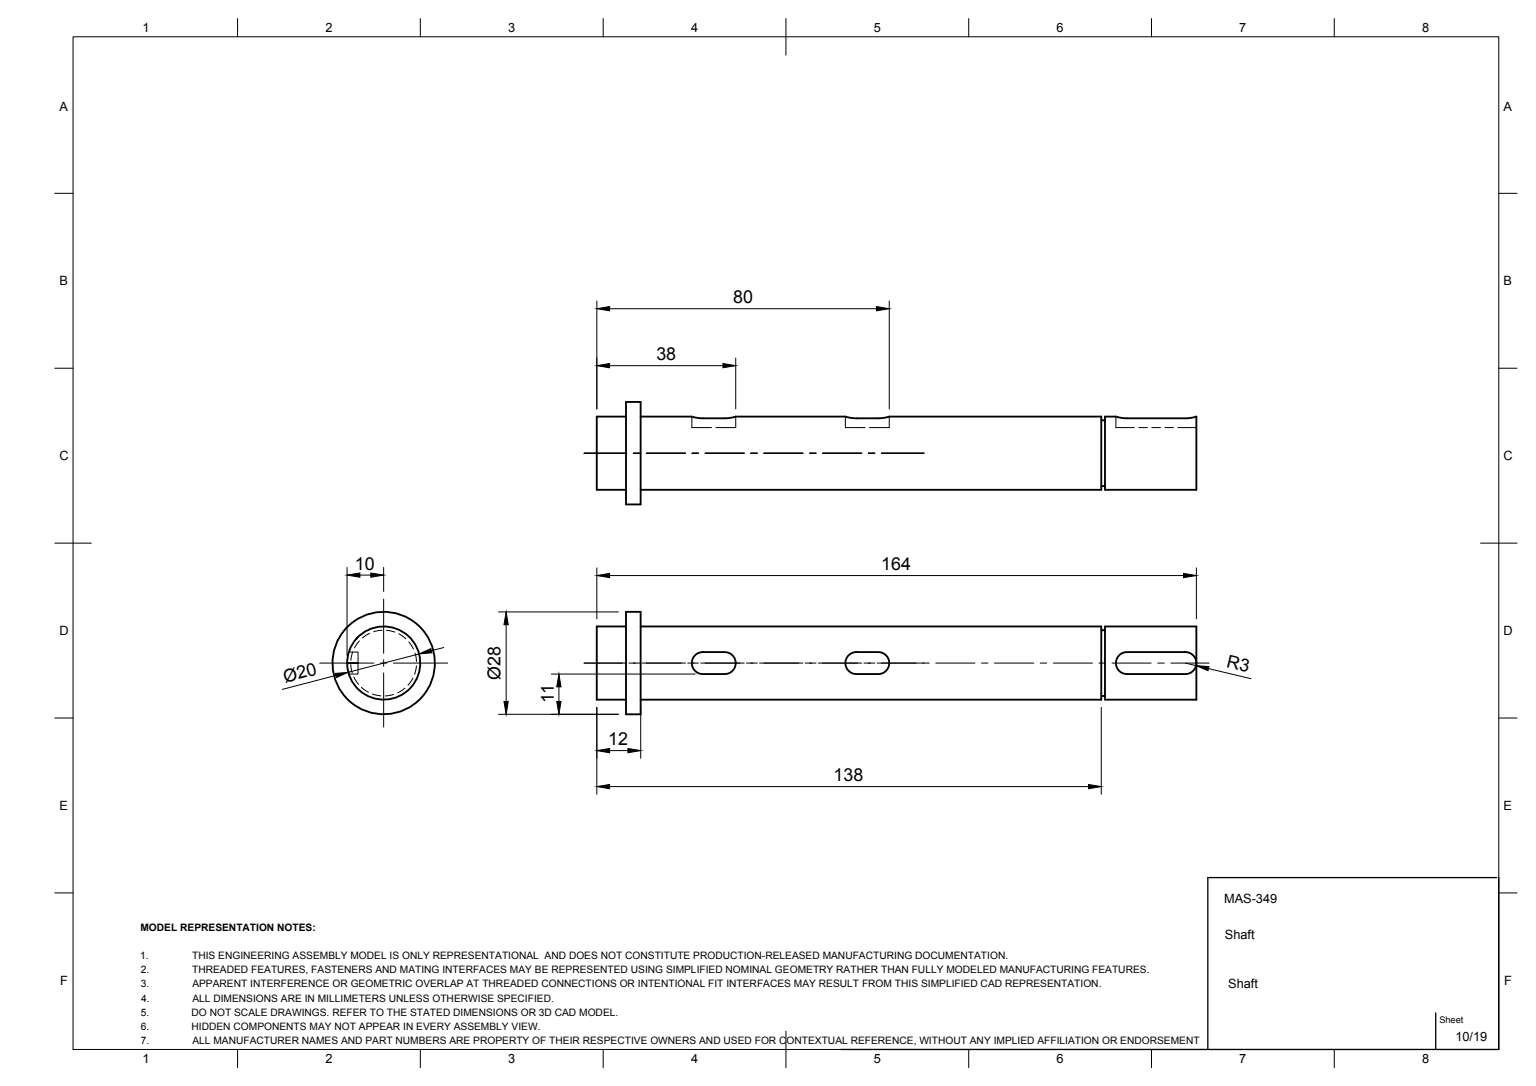
ISO-10303-21;
HEADER;
/* Generated by software containing ST-Developer
 * from STEP Tools, Inc. (www.steptools.com) 
 */

FILE_DESCRIPTION(
/* description */ ('Independent two-stage semi-open centrifugal-pump CAD. Shared impeller
s, open-machinable return casings, removable diaphragms, bronze wear/j
ournal rings, volume-preserving seal instances, retained keyed shaft, 
opposed mechanical face rings and partly threaded tie hardware. Native
 shaft rotation. Geometric topology/clearance only; flow/head/efficien
cy, pressure, cavitation, balance, preload, face loading and secondary
 seal fits/bonds, material/thermal/tolerance selection and life unassi
gned. External drive, coupling, anchors and piping bolts omitted.'),
/* implementation_level */ '2;1');

FILE_NAME(
/* name */ 'Shaft.step',
/* time_stamp */ '2026-11-08T18:06:32-08:00',
/* author */ (''),
/* organization */ (''),
/* preprocessor_version */ 'ST-DEVELOPER v20.2',
/* originating_system */ 'Autodesk Translation Framework v15.17.0.0',
/* authorisation */ '');

FILE_SCHEMA (('AUTOMOTIVE_DESIGN { 1 0 10303 214 3 1 1 }'));
ENDSEC;

DATA;
#10=MECHANICAL_DESIGN_GEOMETRIC_PRESENTATION_REPRESENTATION('',(#400),#16687);
#311=B_SPLINE_CURVE_WITH_KNOTS('',3,(#14886,#14887,#14888,#14889,#14890,
#14891,#14892,#14893,#14894,#14895),.UNSPECIFIED.,.F.,.F.,(4,2,2,2,4),(-0.455064911568752,
-0.341315631981151,-0.227566352393549,-0.113783176196775,0.),
 .UNSPECIFIED.);
#312=B_SPLINE_CURVE_WITH_KNOTS('',3,(#14898,#14899,#14900,#14901,#14902,
#14903,#14904,#14905,#14906,#14907),.UNSPECIFIED.,.F.,.F.,(4,2,2,2,4),(-0.910129823137504,
-0.796346646940729,-0.682563470743954,-0.568814191156353,-0.455064911568752),
 .UNSPECIFIED.);
#313=B_SPLINE_CURVE_WITH_KNOTS('',3,(#14920,#14921,#14922,#14923,#14924,
#14925,#14926,#14927,#14928,#14929,#14930,#14931,#14932,#14933,#14934,#14935,
#14936,#14937),.UNSPECIFIED.,.F.,.F.,(4,2,2,2,2,2,2,2,4),(0.,0.113783176196775,
0.227566352393549,0.34131563198115,0.455064911568751,0.568814191156352,
0.682563470743952,0.796346646940728,0.910129823137503),.UNSPECIFIED.);
#314=B_SPLINE_CURVE_WITH_KNOTS('',3,(#14963,#14964,#14965,#14966,#14967,
#14968,#14969,#14970,#14971,#14972,#14973,#14974,#14975,#14976,#14977,#14978,
#14979,#14980),.UNSPECIFIED.,.F.,.F.,(4,2,2,2,2,2,2,2,4),(-0.910129823137502,
-0.796346646940727,-0.682563470743952,-0.568814191156352,-0.455064911568751,
-0.34131563198115,-0.227566352393549,-0.113783176196775,0.),
 .UNSPECIFIED.);
#315=B_SPLINE_CURVE_WITH_KNOTS('',3,(#14991,#14992,#14993,#14994,#14995,
#14996,#14997,#14998,#14999,#15000,#15001,#15002,#15003,#15004,#15005,#15006,
#15007,#15008),.UNSPECIFIED.,.F.,.F.,(4,2,2,2,2,2,2,2,4),(0.,0.113783176196775,
0.227566352393549,0.34131563198115,0.455064911568751,0.568814191156351,
0.682563470743952,0.796346646940727,0.910129823137502),.UNSPECIFIED.);
#316=B_SPLINE_CURVE_WITH_KNOTS('',3,(#15022,#15023,#15024,#15025,#15026,
#15027,#15028,#15029,#15030,#15031,#15032,#15033,#15034,#15035,#15036,#15037,
#15038,#15039),.UNSPECIFIED.,.F.,.F.,(4,2,2,2,2,2,2,2,4),(-0.910129823137502,
-0.796346646940727,-0.682563470743952,-0.568814191156352,-0.455064911568751,
-0.34131563198115,-0.22756635239355,-0.113783176196775,0.),
 .UNSPECIFIED.);
#317=B_SPLINE_CURVE_WITH_KNOTS('',3,(#15050,#15051,#15052,#15053,#15054,
#15055,#15056,#15057,#15058,#15059,#15060,#15061,#15062,#15063,#15064,#15065,
#15066,#15067),.UNSPECIFIED.,.F.,.F.,(4,2,2,2,2,2,2,2,4),(0.,0.113783176196775,
0.22756635239355,0.341315631981151,0.455064911568751,0.568814191156352,
0.682563470743953,0.796346646940727,0.910129823137502),.UNSPECIFIED.);
#362=SHAPE_REPRESENTATION_RELATIONSHIP('SRR','None',#16771,#381);
#381=ADVANCED_BREP_SHAPE_REPRESENTATION('',(#419),#16675);
#400=STYLED_ITEM('',(#16873),#419);
#419=MANIFOLD_SOLID_BREP('Body1',#6119);
#529=FACE_BOUND('',#1395,.T.);
#530=FACE_BOUND('',#1397,.T.);
#531=FACE_BOUND('',#1399,.T.);
#532=FACE_BOUND('',#1401,.T.);
#533=FACE_BOUND('',#1405,.T.);
#534=FACE_BOUND('',#1406,.T.);
#636=PLANE('',#6783);
#637=PLANE('',#6786);
#638=PLANE('',#6787);
#639=PLANE('',#6792);
#640=PLANE('',#6795);
#641=PLANE('',#6798);
#642=PLANE('',#6799);
#643=PLANE('',#6802);
#644=PLANE('',#6805);
#645=PLANE('',#6809);
#646=PLANE('',#6811);
#647=PLANE('',#6812);
#648=PLANE('',#6815);
#649=PLANE('',#6822);
#650=PLANE('',#6823);
#931=FACE_OUTER_BOUND('',#1376,.T.);
#932=FACE_OUTER_BOUND('',#1377,.T.);
#933=FACE_OUTER_BOUND('',#1378,.T.);
#934=FACE_OUTER_BOUND('',#1379,.T.);
#935=FACE_OUTER_BOUND('',#1380,.T.);
#936=FACE_OUTER_BOUND('',#1381,.T.);
#937=FACE_OUTER_BOUND('',#1382,.T.);
#938=FACE_OUTER_BOUND('',#1383,.T.);
#939=FACE_OUTER_BOUND('',#1384,.T.);
#940=FACE_OUTER_BOUND('',#1385,.T.);
#941=FACE_OUTER_BOUND('',#1386,.T.);
#942=FACE_OUTER_BOUND('',#1387,.T.);
#943=FACE_OUTER_BOUND('',#1388,.T.);
#944=FACE_OUTER_BOUND('',#1389,.T.);
#945=FACE_OUTER_BOUND('',#1390,.T.);
#946=FACE_OUTER_BOUND('',#1391,.T.);
#947=FACE_OUTER_BOUND('',#1392,.T.);
#948=FACE_OUTER_BOUND('',#1393,.T.);
#949=FACE_OUTER_BOUND('',#1394,.T.);
#950=FACE_OUTER_BOUND('',#1396,.T.);
#951=FACE_OUTER_BOUND('',#1398,.T.);
#952=FACE_OUTER_BOUND('',#1400,.T.);
#953=FACE_OUTER_BOUND('',#1402,.T.);
#954=FACE_OUTER_BOUND('',#1403,.T.);
#955=FACE_OUTER_BOUND('',#1404,.T.);
#956=FACE_OUTER_BOUND('',#1407,.T.);
#957=FACE_OUTER_BOUND('',#1408,.T.);
#1376=EDGE_LOOP('',(#5145,#5146,#5147,#5148));
#1377=EDGE_LOOP('',(#5149,#5150,#5151,#5152));
#1378=EDGE_LOOP('',(#5153,#5154,#5155,#5156));
#1379=EDGE_LOOP('',(#5157,#5158,#5159,#5160));
#1380=EDGE_LOOP('',(#5161,#5162,#5163,#5164));
#1381=EDGE_LOOP('',(#5165,#5166,#5167,#5168,#5169));
#1382=EDGE_LOOP('',(#5170,#5171,#5172,#5173,#5174,#5175,#5176,#5177,#5178,
#5179));
#1383=EDGE_LOOP('',(#5180,#5181,#5182,#5183));
#1384=EDGE_LOOP('',(#5184,#5185,#5186,#5187));
#1385=EDGE_LOOP('',(#5188,#5189,#5190,#5191));
#1386=EDGE_LOOP('',(#5192,#5193,#5194,#5195));
#1387=EDGE_LOOP('',(#5196,#5197,#5198,#5199));
#1388=EDGE_LOOP('',(#5200,#5201,#5202,#5203));
#1389=EDGE_LOOP('',(#5204,#5205,#5206,#5207));
#1390=EDGE_LOOP('',(#5208,#5209,#5210,#5211));
#1391=EDGE_LOOP('',(#5212,#5213,#5214,#5215));
#1392=EDGE_LOOP('',(#5216,#5217,#5218,#5219));
#1393=EDGE_LOOP('',(#5220,#5221,#5222,#5223));
#1394=EDGE_LOOP('',(#5224));
#1395=EDGE_LOOP('',(#5225));
#1396=EDGE_LOOP('',(#5226));
#1397=EDGE_LOOP('',(#5227));
#1398=EDGE_LOOP('',(#5228));
#1399=EDGE_LOOP('',(#5229));
#1400=EDGE_LOOP('',(#5230));
#1401=EDGE_LOOP('',(#5231));
#1402=EDGE_LOOP('',(#5232,#5233,#5234,#5235));
#1403=EDGE_LOOP('',(#5236,#5237,#5238,#5239));
#1404=EDGE_LOOP('',(#5240,#5241,#5242,#5243));
#1405=EDGE_LOOP('',(#5244,#5245,#5246,#5247));
#1406=EDGE_LOOP('',(#5248,#5249,#5250,#5251));
#1407=EDGE_LOOP('',(#5252,#5253,#5254,#5255));
#1408=EDGE_LOOP('',(#5256));
#1773=LINE('',#14881,#2142);
#1774=LINE('',#14885,#2143);
#1775=LINE('',#14909,#2144);
#1776=LINE('',#14911,#2145);
#1777=LINE('',#14914,#2146);
#1778=LINE('',#14916,#2147);
#1779=LINE('',#14917,#2148);
#1780=LINE('',#14940,#2149);
#1781=LINE('',#14942,#2150);
#1782=LINE('',#14943,#2151);
#1783=LINE('',#14950,#2152);
#1784=LINE('',#14955,#2153);
#1785=LINE('',#14957,#2154);
#1786=LINE('',#14959,#2155);
#1787=LINE('',#14960,#2156);
#1788=LINE('',#14983,#2157);
#1789=LINE('',#14986,#2158);
#1790=LINE('',#14988,#2159);
#1791=LINE('',#14989,#2160);
#1792=LINE('',#15014,#2161);
#1793=LINE('',#15016,#2162);
#1794=LINE('',#15018,#2163);
#1795=LINE('',#15019,#2164);
#1796=LINE('',#15042,#2165);
#1797=LINE('',#15045,#2166);
#1798=LINE('',#15047,#2167);
#1799=LINE('',#15048,#2168);
#1800=LINE('',#15074,#2169);
#1801=LINE('',#15091,#2170);
#1802=LINE('',#15094,#2171);
#1803=LINE('',#15097,#2172);
#2142=VECTOR('',#8137,1.);
#2143=VECTOR('',#8140,1.);
#2144=VECTOR('',#8143,1.);
#2145=VECTOR('',#8146,1.);
#2146=VECTOR('',#8149,1.);
#2147=VECTOR('',#8150,1.);
#2148=VECTOR('',#8151,1.);
#2149=VECTOR('',#8156,1.);
#2150=VECTOR('',#8159,1.);
#2151=VECTOR('',#8160,1.);
#2152=VECTOR('',#8169,1.);
#2153=VECTOR('',#8174,1.);
#2154=VECTOR('',#8175,1.);
#2155=VECTOR('',#8176,1.);
#2156=VECTOR('',#8177,1.);
#2157=VECTOR('',#8182,1.);
#2158=VECTOR('',#8185,1.);
#2159=VECTOR('',#8186,1.);
#2160=VECTOR('',#8187,1.);
#2161=VECTOR('',#8196,1.);
#2162=VECTOR('',#8197,1.);
#2163=VECTOR('',#8198,1.);
#2164=VECTOR('',#8199,1.);
#2165=VECTOR('',#8204,1.);
#2166=VECTOR('',#8207,1.);
#2167=VECTOR('',#8208,1.);
#2168=VECTOR('',#8209,1.);
#2169=VECTOR('',#8220,0.9);
#2170=VECTOR('',#8243,1.4);
#2171=VECTOR('',#8246,1.);
#2172=VECTOR('',#8251,1.);
#2432=CIRCLE('',#6780,0.3);
#2433=CIRCLE('',#6782,0.3);
#2434=CIRCLE('',#6785,0.3);
#2435=CIRCLE('',#6789,1.);
#2436=CIRCLE('',#6790,1.);
#2437=CIRCLE('',#6791,1.);
#2438=CIRCLE('',#6794,0.3);
#2439=CIRCLE('',#6797,0.3);
#2440=CIRCLE('',#6801,0.3);
#2441=CIRCLE('',#6804,0.3);
#2442=CIRCLE('',#6807,0.9);
#2443=CIRCLE('',#6808,0.9);
#2444=CIRCLE('',#6810,1.);
#2445=CIRCLE('',#6813,1.4);
#2446=CIRCLE('',#6814,1.);
#2447=CIRCLE('',#6816,1.4);
#2448=CIRCLE('',#6817,1.);
#2449=CIRCLE('',#6820,1.);
#2917=VERTEX_POINT('',#14879);
#2918=VERTEX_POINT('',#14880);
#2919=VERTEX_POINT('',#14882);
#2920=VERTEX_POINT('',#14884);
#2921=VERTEX_POINT('',#14897);
#2922=VERTEX_POINT('',#14908);
#2923=VERTEX_POINT('',#14913);
#2924=VERTEX_POINT('',#14915);
#2925=VERTEX_POINT('',#14919);
#2926=VERTEX_POINT('',#14938);
#2927=VERTEX_POINT('',#14946);
#2928=VERTEX_POINT('',#14949);
#2929=VERTEX_POINT('',#14953);
#2930=VERTEX_POINT('',#14954);
#2931=VERTEX_POINT('',#14956);
#2932=VERTEX_POINT('',#14958);
#2933=VERTEX_POINT('',#14962);
#2934=VERTEX_POINT('',#14981);
#2935=VERTEX_POINT('',#14985);
#2936=VERTEX_POINT('',#14987);
#2937=VERTEX_POINT('',#15012);
#2938=VERTEX_POINT('',#15013);
#2939=VERTEX_POINT('',#15015);
#2940=VERTEX_POINT('',#15017);
#2941=VERTEX_POINT('',#15021);
#2942=VERTEX_POINT('',#15040);
#2943=VERTEX_POINT('',#15044);
#2944=VERTEX_POINT('',#15046);
#2945=VERTEX_POINT('',#15071);
#2946=VERTEX_POINT('',#15073);
#2947=VERTEX_POINT('',#15077);
#2948=VERTEX_POINT('',#15081);
#2949=VERTEX_POINT('',#15083);
#2950=VERTEX_POINT('',#15086);
#2951=VERTEX_POINT('',#15088);
#2952=VERTEX_POINT('',#15093);
#3682=EDGE_CURVE('',#2917,#2918,#1773,.T.);
#3683=EDGE_CURVE('',#2919,#2917,#2432,.T.);
#3684=EDGE_CURVE('',#2919,#2920,#1774,.T.);
#3685=EDGE_CURVE('',#2918,#2920,#311,.T.);
#3686=EDGE_CURVE('',#2921,#2918,#312,.T.);
#3687=EDGE_CURVE('',#2922,#2921,#1775,.T.);
#3688=EDGE_CURVE('',#2917,#2922,#2433,.T.);
#3689=EDGE_CURVE('',#2917,#2918,#1776,.T.);
#3690=EDGE_CURVE('',#2920,#2923,#1777,.T.);
#3691=EDGE_CURVE('',#2919,#2924,#1778,.T.);
#3692=EDGE_CURVE('',#2924,#2923,#1779,.T.);
#3693=EDGE_CURVE('',#2923,#2925,#313,.T.);
#3694=EDGE_CURVE('',#2926,#2924,#2434,.T.);
#3695=EDGE_CURVE('',#2926,#2925,#1780,.T.);
#3696=EDGE_CURVE('',#2925,#2921,#1781,.T.);
#3697=EDGE_CURVE('',#2926,#2922,#1782,.T.);
#3698=EDGE_CURVE('',#2918,#2927,#2435,.T.);
#3699=EDGE_CURVE('',#2927,#2918,#2436,.T.);
#3700=EDGE_CURVE('',#2927,#2928,#1783,.T.);
#3701=EDGE_CURVE('',#2928,#2928,#2437,.T.);
#3702=EDGE_CURVE('',#2929,#2930,#1784,.T.);
#3703=EDGE_CURVE('',#2931,#2929,#1785,.T.);
#3704=EDGE_CURVE('',#2931,#2932,#1786,.T.);
#3705=EDGE_CURVE('',#2932,#2930,#1787,.T.);
#3706=EDGE_CURVE('',#2930,#2933,#314,.T.);
#3707=EDGE_CURVE('',#2934,#2932,#2438,.T.);
#3708=EDGE_CURVE('',#2934,#2933,#1788,.T.);
#3709=EDGE_CURVE('',#2933,#2935,#1789,.T.);
#3710=EDGE_CURVE('',#2934,#2936,#1790,.T.);
#3711=EDGE_CURVE('',#2936,#2935,#1791,.T.);
#3712=EDGE_CURVE('',#2935,#2929,#315,.T.);
#3713=EDGE_CURVE('',#2931,#2936,#2439,.T.);
#3714=EDGE_CURVE('',#2937,#2938,#1792,.T.);
#3715=EDGE_CURVE('',#2939,#2937,#1793,.T.);
#3716=EDGE_CURVE('',#2939,#2940,#1794,.T.);
#3717=EDGE_CURVE('',#2940,#2938,#1795,.T.);
#3718=EDGE_CURVE('',#2938,#2941,#316,.T.);
#3719=EDGE_CURVE('',#2942,#2940,#2440,.T.);
#3720=EDGE_CURVE('',#2942,#2941,#1796,.T.);
#3721=EDGE_CURVE('',#2941,#2943,#1797,.T.);
#3722=EDGE_CURVE('',#2942,#2944,#1798,.T.);
#3723=EDGE_CURVE('',#2944,#2943,#1799,.T.);
#3724=EDGE_CURVE('',#2943,#2937,#317,.T.);
#3725=EDGE_CURVE('',#2939,#2944,#2441,.T.);
#3726=EDGE_CURVE('',#2945,#2945,#2442,.T.);
#3727=EDGE_CURVE('',#2945,#2946,#1800,.T.);
#3728=EDGE_CURVE('',#2946,#2946,#2443,.T.);
#3729=EDGE_CURVE('',#2947,#2947,#2444,.T.);
#3730=EDGE_CURVE('',#2948,#2948,#2445,.T.);
#3731=EDGE_CURVE('',#2949,#2949,#2446,.T.);
#3732=EDGE_CURVE('',#2950,#2950,#2447,.T.);
#3733=EDGE_CURVE('',#2951,#2951,#2448,.T.);
#3734=EDGE_CURVE('',#2948,#2950,#1801,.T.);
#3735=EDGE_CURVE('',#2951,#2952,#1802,.T.);
#3736=EDGE_CURVE('',#2952,#2952,#2449,.T.);
#3737=EDGE_CURVE('',#2947,#2949,#1803,.T.);
#5145=ORIENTED_EDGE('',*,*,#3682,.F.);
#5146=ORIENTED_EDGE('',*,*,#3683,.F.);
#5147=ORIENTED_EDGE('',*,*,#3684,.T.);
#5148=ORIENTED_EDGE('',*,*,#3685,.F.);
#5149=ORIENTED_EDGE('',*,*,#3686,.F.);
#5150=ORIENTED_EDGE('',*,*,#3687,.F.);
#5151=ORIENTED_EDGE('',*,*,#3688,.F.);
#5152=ORIENTED_EDGE('',*,*,#3689,.T.);
#5153=ORIENTED_EDGE('',*,*,#3690,.F.);
#5154=ORIENTED_EDGE('',*,*,#3684,.F.);
#5155=ORIENTED_EDGE('',*,*,#3691,.T.);
#5156=ORIENTED_EDGE('',*,*,#3692,.T.);
#5157=ORIENTED_EDGE('',*,*,#3693,.F.);
#5158=ORIENTED_EDGE('',*,*,#3692,.F.);
#5159=ORIENTED_EDGE('',*,*,#3694,.F.);
#5160=ORIENTED_EDGE('',*,*,#3695,.T.);
#5161=ORIENTED_EDGE('',*,*,#3696,.F.);
#5162=ORIENTED_EDGE('',*,*,#3695,.F.);
#5163=ORIENTED_EDGE('',*,*,#3697,.T.);
#5164=ORIENTED_EDGE('',*,*,#3687,.T.);
#5165=ORIENTED_EDGE('',*,*,#3683,.T.);
#5166=ORIENTED_EDGE('',*,*,#3688,.T.);
#5167=ORIENTED_EDGE('',*,*,#3697,.F.);
#5168=ORIENTED_EDGE('',*,*,#3694,.T.);
#5169=ORIENTED_EDGE('',*,*,#3691,.F.);
#5170=ORIENTED_EDGE('',*,*,#3698,.F.);
#5171=ORIENTED_EDGE('',*,*,#3685,.T.);
#5172=ORIENTED_EDGE('',*,*,#3690,.T.);
#5173=ORIENTED_EDGE('',*,*,#3693,.T.);
#5174=ORIENTED_EDGE('',*,*,#3696,.T.);
#5175=ORIENTED_EDGE('',*,*,#3686,.T.);
#5176=ORIENTED_EDGE('',*,*,#3699,.F.);
#5177=ORIENTED_EDGE('',*,*,#3700,.T.);
#5178=ORIENTED_EDGE('',*,*,#3701,.T.);
#5179=ORIENTED_EDGE('',*,*,#3700,.F.);
#5180=ORIENTED_EDGE('',*,*,#3702,.F.);
#5181=ORIENTED_EDGE('',*,*,#3703,.F.);
#5182=ORIENTED_EDGE('',*,*,#3704,.T.);
#5183=ORIENTED_EDGE('',*,*,#3705,.T.);
#5184=ORIENTED_EDGE('',*,*,#3706,.F.);
#5185=ORIENTED_EDGE('',*,*,#3705,.F.);
#5186=ORIENTED_EDGE('',*,*,#3707,.F.);
#5187=ORIENTED_EDGE('',*,*,#3708,.T.);
#5188=ORIENTED_EDGE('',*,*,#3709,.F.);
#5189=ORIENTED_EDGE('',*,*,#3708,.F.);
#5190=ORIENTED_EDGE('',*,*,#3710,.T.);
#5191=ORIENTED_EDGE('',*,*,#3711,.T.);
#5192=ORIENTED_EDGE('',*,*,#3712,.F.);
#5193=ORIENTED_EDGE('',*,*,#3711,.F.);
#5194=ORIENTED_EDGE('',*,*,#3713,.F.);
#5195=ORIENTED_EDGE('',*,*,#3703,.T.);
#5196=ORIENTED_EDGE('',*,*,#3707,.T.);
#5197=ORIENTED_EDGE('',*,*,#3704,.F.);
#5198=ORIENTED_EDGE('',*,*,#3713,.T.);
#5199=ORIENTED_EDGE('',*,*,#3710,.F.);
#5200=ORIENTED_EDGE('',*,*,#3714,.F.);
#5201=ORIENTED_EDGE('',*,*,#3715,.F.);
#5202=ORIENTED_EDGE('',*,*,#3716,.T.);
#5203=ORIENTED_EDGE('',*,*,#3717,.T.);
#5204=ORIENTED_EDGE('',*,*,#3718,.F.);
#5205=ORIENTED_EDGE('',*,*,#3717,.F.);
#5206=ORIENTED_EDGE('',*,*,#3719,.F.);
#5207=ORIENTED_EDGE('',*,*,#3720,.T.);
#5208=ORIENTED_EDGE('',*,*,#3721,.F.);
#5209=ORIENTED_EDGE('',*,*,#3720,.F.);
#5210=ORIENTED_EDGE('',*,*,#3722,.T.);
#5211=ORIENTED_EDGE('',*,*,#3723,.T.);
#5212=ORIENTED_EDGE('',*,*,#3724,.F.);
#5213=ORIENTED_EDGE('',*,*,#3723,.F.);
#5214=ORIENTED_EDGE('',*,*,#3725,.F.);
#5215=ORIENTED_EDGE('',*,*,#3715,.T.);
#5216=ORIENTED_EDGE('',*,*,#3719,.T.);
#5217=ORIENTED_EDGE('',*,*,#3716,.F.);
#5218=ORIENTED_EDGE('',*,*,#3725,.T.);
#5219=ORIENTED_EDGE('',*,*,#3722,.F.);
#5220=ORIENTED_EDGE('',*,*,#3726,.T.);
#5221=ORIENTED_EDGE('',*,*,#3727,.T.);
#5222=ORIENTED_EDGE('',*,*,#3728,.F.);
#5223=ORIENTED_EDGE('',*,*,#3727,.F.);
#5224=ORIENTED_EDGE('',*,*,#3729,.F.);
#5225=ORIENTED_EDGE('',*,*,#3726,.F.);
#5226=ORIENTED_EDGE('',*,*,#3701,.F.);
#5227=ORIENTED_EDGE('',*,*,#3728,.T.);
#5228=ORIENTED_EDGE('',*,*,#3730,.T.);
#5229=ORIENTED_EDGE('',*,*,#3731,.F.);
#5230=ORIENTED_EDGE('',*,*,#3732,.F.);
#5231=ORIENTED_EDGE('',*,*,#3733,.F.);
#5232=ORIENTED_EDGE('',*,*,#3730,.F.);
#5233=ORIENTED_EDGE('',*,*,#3734,.T.);
#5234=ORIENTED_EDGE('',*,*,#3732,.T.);
#5235=ORIENTED_EDGE('',*,*,#3734,.F.);
#5236=ORIENTED_EDGE('',*,*,#3733,.T.);
#5237=ORIENTED_EDGE('',*,*,#3735,.T.);
#5238=ORIENTED_EDGE('',*,*,#3736,.T.);
#5239=ORIENTED_EDGE('',*,*,#3735,.F.);
#5240=ORIENTED_EDGE('',*,*,#3729,.T.);
#5241=ORIENTED_EDGE('',*,*,#3737,.T.);
#5242=ORIENTED_EDGE('',*,*,#3731,.T.);
#5243=ORIENTED_EDGE('',*,*,#3737,.F.);
#5244=ORIENTED_EDGE('',*,*,#3709,.T.);
#5245=ORIENTED_EDGE('',*,*,#3712,.T.);
#5246=ORIENTED_EDGE('',*,*,#3702,.T.);
#5247=ORIENTED_EDGE('',*,*,#3706,.T.);
#5248=ORIENTED_EDGE('',*,*,#3721,.T.);
#5249=ORIENTED_EDGE('',*,*,#3724,.T.);
#5250=ORIENTED_EDGE('',*,*,#3714,.T.);
#5251=ORIENTED_EDGE('',*,*,#3718,.T.);
#5252=ORIENTED_EDGE('',*,*,#3698,.T.);
#5253=ORIENTED_EDGE('',*,*,#3699,.T.);
#5254=ORIENTED_EDGE('',*,*,#3689,.F.);
#5255=ORIENTED_EDGE('',*,*,#3682,.T.);
#5256=ORIENTED_EDGE('',*,*,#3736,.F.);
#5716=CYLINDRICAL_SURFACE('',#6779,0.3);
#5717=CYLINDRICAL_SURFACE('',#6781,0.3);
#5718=CYLINDRICAL_SURFACE('',#6784,0.3);
#5719=CYLINDRICAL_SURFACE('',#6788,1.);
#5720=CYLINDRICAL_SURFACE('',#6793,0.3);
#5721=CYLINDRICAL_SURFACE('',#6796,0.3);
#5722=CYLINDRICAL_SURFACE('',#6800,0.3);
#5723=CYLINDRICAL_SURFACE('',#6803,0.3);
#5724=CYLINDRICAL_SURFACE('',#6806,0.9);
#5725=CYLINDRICAL_SURFACE('',#6818,1.4);
#5726=CYLINDRICAL_SURFACE('',#6819,1.);
#5727=CYLINDRICAL_SURFACE('',#6821,1.);
#6010=ADVANCED_FACE('',(#931),#5716,.F.);
#6011=ADVANCED_FACE('',(#932),#5717,.F.);
#6012=ADVANCED_FACE('',(#933),#636,.F.);
#6013=ADVANCED_FACE('',(#934),#5718,.F.);
#6014=ADVANCED_FACE('',(#935),#637,.F.);
#6015=ADVANCED_FACE('',(#936),#638,.T.);
#6016=ADVANCED_FACE('',(#937),#5719,.T.);
#6017=ADVANCED_FACE('',(#938),#639,.F.);
#6018=ADVANCED_FACE('',(#939),#5720,.F.);
#6019=ADVANCED_FACE('',(#940),#640,.F.);
#6020=ADVANCED_FACE('',(#941),#5721,.F.);
#6021=ADVANCED_FACE('',(#942),#641,.T.);
#6022=ADVANCED_FACE('',(#943),#642,.F.);
#6023=ADVANCED_FACE('',(#944),#5722,.F.);
#6024=ADVANCED_FACE('',(#945),#643,.F.);
#6025=ADVANCED_FACE('',(#946),#5723,.F.);
#6026=ADVANCED_FACE('',(#947),#644,.T.);
#6027=ADVANCED_FACE('',(#948),#5724,.T.);
#6028=ADVANCED_FACE('',(#949,#529),#645,.F.);
#6029=ADVANCED_FACE('',(#950,#530),#646,.F.);
#6030=ADVANCED_FACE('',(#951,#531),#647,.T.);
#6031=ADVANCED_FACE('',(#952,#532),#648,.F.);
#6032=ADVANCED_FACE('',(#953),#5725,.T.);
#6033=ADVANCED_FACE('',(#954),#5726,.T.);
#6034=ADVANCED_FACE('',(#955,#533,#534),#5727,.T.);
#6035=ADVANCED_FACE('',(#956),#649,.T.);
#6036=ADVANCED_FACE('',(#957),#650,.F.);
#6119=CLOSED_SHELL('',(#6010,#6011,#6012,#6013,#6014,#6015,#6016,#6017,
#6018,#6019,#6020,#6021,#6022,#6023,#6024,#6025,#6026,#6027,#6028,#6029,
#6030,#6031,#6032,#6033,#6034,#6035,#6036));
#6778=AXIS2_PLACEMENT_3D('',#14877,#8133,#8134);
#6779=AXIS2_PLACEMENT_3D('',#14878,#8135,#8136);
#6780=AXIS2_PLACEMENT_3D('',#14883,#8138,#8139);
#6781=AXIS2_PLACEMENT_3D('',#14896,#8141,#8142);
#6782=AXIS2_PLACEMENT_3D('',#14910,#8144,#8145);
#6783=AXIS2_PLACEMENT_3D('',#14912,#8147,#8148);
#6784=AXIS2_PLACEMENT_3D('',#14918,#8152,#8153);
#6785=AXIS2_PLACEMENT_3D('',#14939,#8154,#8155);
#6786=AXIS2_PLACEMENT_3D('',#14941,#8157,#8158);
#6787=AXIS2_PLACEMENT_3D('',#14944,#8161,#8162);
#6788=AXIS2_PLACEMENT_3D('',#14945,#8163,#8164);
#6789=AXIS2_PLACEMENT_3D('',#14947,#8165,#8166);
#6790=AXIS2_PLACEMENT_3D('',#14948,#8167,#8168);
#6791=AXIS2_PLACEMENT_3D('',#14951,#8170,#8171);
#6792=AXIS2_PLACEMENT_3D('',#14952,#8172,#8173);
#6793=AXIS2_PLACEMENT_3D('',#14961,#8178,#8179);
#6794=AXIS2_PLACEMENT_3D('',#14982,#8180,#8181);
#6795=AXIS2_PLACEMENT_3D('',#14984,#8183,#8184);
#6796=AXIS2_PLACEMENT_3D('',#14990,#8188,#8189);
#6797=AXIS2_PLACEMENT_3D('',#15009,#8190,#8191);
#6798=AXIS2_PLACEMENT_3D('',#15010,#8192,#8193);
#6799=AXIS2_PLACEMENT_3D('',#15011,#8194,#8195);
#6800=AXIS2_PLACEMENT_3D('',#15020,#8200,#8201);
#6801=AXIS2_PLACEMENT_3D('',#15041,#8202,#8203);
#6802=AXIS2_PLACEMENT_3D('',#15043,#8205,#8206);
#6803=AXIS2_PLACEMENT_3D('',#15049,#8210,#8211);
#6804=AXIS2_PLACEMENT_3D('',#15068,#8212,#8213);
#6805=AXIS2_PLACEMENT_3D('',#15069,#8214,#8215);
#6806=AXIS2_PLACEMENT_3D('',#15070,#8216,#8217);
#6807=AXIS2_PLACEMENT_3D('',#15072,#8218,#8219);
#6808=AXIS2_PLACEMENT_3D('',#15075,#8221,#8222);
#6809=AXIS2_PLACEMENT_3D('',#15076,#8223,#8224);
#6810=AXIS2_PLACEMENT_3D('',#15078,#8225,#8226);
#6811=AXIS2_PLACEMENT_3D('',#15079,#8227,#8228);
#6812=AXIS2_PLACEMENT_3D('',#15080,#8229,#8230);
#6813=AXIS2_PLACEMENT_3D('',#15082,#8231,#8232);
#6814=AXIS2_PLACEMENT_3D('',#15084,#8233,#8234);
#6815=AXIS2_PLACEMENT_3D('',#15085,#8235,#8236);
#6816=AXIS2_PLACEMENT_3D('',#15087,#8237,#8238);
#6817=AXIS2_PLACEMENT_3D('',#15089,#8239,#8240);
#6818=AXIS2_PLACEMENT_3D('',#15090,#8241,#8242);
#6819=AXIS2_PLACEMENT_3D('',#15092,#8244,#8245);
#6820=AXIS2_PLACEMENT_3D('',#15095,#8247,#8248);
#6821=AXIS2_PLACEMENT_3D('',#15096,#8249,#8250);
#6822=AXIS2_PLACEMENT_3D('',#15098,#8252,#8253);
#6823=AXIS2_PLACEMENT_3D('',#15099,#8254,#8255);
#8133=DIRECTION('axis',(0.,0.,1.));
#8134=DIRECTION('refdir',(1.,0.,0.));
#8135=DIRECTION('center_axis',(1.,0.,0.));
#8136=DIRECTION('ref_axis',(0.,1.,5.9211894646675E-15));
#8137=DIRECTION('',(1.,0.,0.));
#8138=DIRECTION('center_axis',(1.,0.,0.));
#8139=DIRECTION('ref_axis',(0.,1.,5.9211894646675E-15));
#8140=DIRECTION('',(1.,0.,0.));
#8141=DIRECTION('center_axis',(1.,0.,0.));
#8142=DIRECTION('ref_axis',(0.,1.,5.9211894646675E-15));
#8143=DIRECTION('',(1.,0.,0.));
#8144=DIRECTION('center_axis',(1.,0.,0.));
#8145=DIRECTION('ref_axis',(0.,1.,5.9211894646675E-15));
#8146=DIRECTION('',(1.,0.,0.));
#8147=DIRECTION('center_axis',(0.,1.,0.));
#8148=DIRECTION('ref_axis',(0.,0.,1.));
#8149=DIRECTION('',(0.,0.,-1.));
#8150=DIRECTION('',(0.,0.,-1.));
#8151=DIRECTION('',(1.,0.,0.));
#8152=DIRECTION('center_axis',(1.,0.,0.));
#8153=DIRECTION('ref_axis',(0.,-1.,-5.9211894646675E-15));
#8154=DIRECTION('center_axis',(1.,0.,0.));
#8155=DIRECTION('ref_axis',(0.,-1.,-5.9211894646675E-15));
#8156=DIRECTION('',(1.,0.,0.));
#8157=DIRECTION('center_axis',(0.,-1.,0.));
#8158=DIRECTION('ref_axis',(0.,0.,-1.));
#8159=DIRECTION('',(0.,0.,1.));
#8160=DIRECTION('',(0.,0.,1.));
#8161=DIRECTION('center_axis',(1.,0.,0.));
#8162=DIRECTION('ref_axis',(0.,0.,-1.));
#8163=DIRECTION('center_axis',(0.,0.,1.));
#8164=DIRECTION('ref_axis',(1.,0.,0.));
#8165=DIRECTION('center_axis',(0.,0.,1.));
#8166=DIRECTION('ref_axis',(1.,0.,0.));
#8167=DIRECTION('center_axis',(0.,0.,1.));
#8168=DIRECTION('ref_axis',(1.,0.,0.));
#8169=DIRECTION('',(0.,0.,-1.));
#8170=DIRECTION('center_axis',(0.,0.,1.));
#8171=DIRECTION('ref_axis',(1.,0.,0.));
#8172=DIRECTION('center_axis',(0.,-1.,0.));
#8173=DIRECTION('ref_axis',(0.,0.,-1.));
#8174=DIRECTION('',(0.,0.,1.));
#8175=DIRECTION('',(1.,0.,0.));
#8176=DIRECTION('',(0.,0.,1.));
#8177=DIRECTION('',(1.,0.,0.));
#8178=DIRECTION('center_axis',(1.,0.,0.));
#8179=DIRECTION('ref_axis',(0.,1.,0.));
#8180=DIRECTION('center_axis',(1.,0.,0.));
#8181=DIRECTION('ref_axis',(0.,1.,0.));
#8182=DIRECTION('',(1.,0.,0.));
#8183=DIRECTION('center_axis',(0.,1.,0.));
#8184=DIRECTION('ref_axis',(0.,0.,1.));
#8185=DIRECTION('',(0.,0.,-1.));
#8186=DIRECTION('',(0.,0.,-1.));
#8187=DIRECTION('',(1.,0.,0.));
#8188=DIRECTION('center_axis',(1.,0.,0.));
#8189=DIRECTION('ref_axis',(0.,-1.,-2.96059473233375E-15));
#8190=DIRECTION('center_axis',(1.,0.,0.));
#8191=DIRECTION('ref_axis',(0.,-1.,-2.96059473233375E-15));
#8192=DIRECTION('center_axis',(1.,0.,0.));
#8193=DIRECTION('ref_axis',(0.,0.,-1.));
#8194=DIRECTION('center_axis',(0.,-1.,0.));
#8195=DIRECTION('ref_axis',(0.,0.,-1.));
#8196=DIRECTION('',(0.,0.,1.));
#8197=DIRECTION('',(1.,0.,0.));
#8198=DIRECTION('',(0.,0.,1.));
#8199=DIRECTION('',(1.,0.,0.));
#8200=DIRECTION('center_axis',(1.,0.,0.));
#8201=DIRECTION('ref_axis',(0.,1.,0.));
#8202=DIRECTION('center_axis',(1.,0.,0.));
#8203=DIRECTION('ref_axis',(0.,1.,0.));
#8204=DIRECTION('',(1.,0.,0.));
#8205=DIRECTION('center_axis',(0.,1.,0.));
#8206=DIRECTION('ref_axis',(0.,0.,1.));
#8207=DIRECTION('',(0.,0.,-1.));
#8208=DIRECTION('',(0.,0.,-1.));
#8209=DIRECTION('',(1.,0.,0.));
#8210=DIRECTION('center_axis',(1.,0.,0.));
#8211=DIRECTION('ref_axis',(0.,-1.,0.));
#8212=DIRECTION('center_axis',(1.,0.,0.));
#8213=DIRECTION('ref_axis',(0.,-1.,0.));
#8214=DIRECTION('center_axis',(1.,0.,0.));
#8215=DIRECTION('ref_axis',(0.,0.,-1.));
#8216=DIRECTION('center_axis',(0.,0.,1.));
#8217=DIRECTION('ref_axis',(1.,0.,0.));
#8218=DIRECTION('center_axis',(0.,0.,1.));
#8219=DIRECTION('ref_axis',(1.,0.,0.));
#8220=DIRECTION('',(0.,0.,1.));
#8221=DIRECTION('center_axis',(0.,0.,1.));
#8222=DIRECTION('ref_axis',(1.,0.,0.));
#8223=DIRECTION('center_axis',(0.,0.,-1.));
#8224=DIRECTION('ref_axis',(-1.,0.,0.));
#8225=DIRECTION('center_axis',(0.,0.,-1.));
#8226=DIRECTION('ref_axis',(1.,0.,0.));
#8227=DIRECTION('center_axis',(0.,0.,1.));
#8228=DIRECTION('ref_axis',(1.,0.,0.));
#8229=DIRECTION('center_axis',(0.,0.,1.));
#8230=DIRECTION('ref_axis',(1.,0.,0.));
#8231=DIRECTION('center_axis',(0.,0.,1.));
#8232=DIRECTION('ref_axis',(1.,0.,0.));
#8233=DIRECTION('center_axis',(0.,0.,1.));
#8234=DIRECTION('ref_axis',(1.,0.,0.));
#8235=DIRECTION('center_axis',(0.,0.,1.));
#8236=DIRECTION('ref_axis',(1.,0.,0.));
#8237=DIRECTION('center_axis',(0.,0.,1.));
#8238=DIRECTION('ref_axis',(1.,0.,0.));
#8239=DIRECTION('center_axis',(0.,0.,-1.));
#8240=DIRECTION('ref_axis',(1.,0.,0.));
#8241=DIRECTION('center_axis',(0.,0.,1.));
#8242=DIRECTION('ref_axis',(1.,0.,0.));
#8243=DIRECTION('',(0.,0.,-1.));
#8244=DIRECTION('center_axis',(0.,0.,1.));
#8245=DIRECTION('ref_axis',(1.,0.,0.));
#8246=DIRECTION('',(0.,0.,-1.));
#8247=DIRECTION('center_axis',(0.,0.,1.));
#8248=DIRECTION('ref_axis',(1.,0.,0.));
#8249=DIRECTION('center_axis',(0.,0.,1.));
#8250=DIRECTION('ref_axis',(1.,0.,0.));
#8251=DIRECTION('',(0.,0.,-1.));
#8252=DIRECTION('center_axis',(0.,0.,1.));
#8253=DIRECTION('ref_axis',(1.,0.,0.));
#8254=DIRECTION('center_axis',(0.,0.,1.));
#8255=DIRECTION('ref_axis',(1.,0.,0.));
#14877=CARTESIAN_POINT('',(0.,0.,0.));
#14878=CARTESIAN_POINT('Origin',(0.7,0.,15.3));
#14879=CARTESIAN_POINT('',(0.7,0.,15.6));
#14880=CARTESIAN_POINT('',(1.,0.,15.6));
#14881=CARTESIAN_POINT('',(0.7,0.,15.6));
#14882=CARTESIAN_POINT('',(0.7,0.3,15.3));
#14883=CARTESIAN_POINT('Origin',(0.7,0.,15.3));
#14884=CARTESIAN_POINT('',(0.953939201416946,0.3,15.3));
#14885=CARTESIAN_POINT('',(0.7,0.3,15.3));
#14886=CARTESIAN_POINT('Ctrl Pts',(1.,-3.88578058618805E-16,15.6));
#14887=CARTESIAN_POINT('Ctrl Pts',(1.,0.0379164265292001,15.6));
#14888=CARTESIAN_POINT('Ctrl Pts',(0.997630133387832,0.0782037717481895,
15.5923748246511));
#14889=CARTESIAN_POINT('Ctrl Pts',(0.989071194990079,0.152052241900625,
15.5616848907033));
#14890=CARTESIAN_POINT('Ctrl Pts',(0.982993562614982,0.185631434471708,
15.5386326342402));
#14891=CARTESIAN_POINT('Ctrl Pts',(0.971486751729016,0.238640531261463,
15.4856235374505));
#14892=CARTESIAN_POINT('Ctrl Pts',(0.965284956103207,0.261686672615768,
15.4520475537716));
#14893=CARTESIAN_POINT('Ctrl Pts',(0.956437939057487,0.292372091609923,
15.3782107485428));
#14894=CARTESIAN_POINT('Ctrl Pts',(0.953939201416946,0.3,15.3379277253989));
#14895=CARTESIAN_POINT('Ctrl Pts',(0.953939201416946,0.3,15.3));
#14896=CARTESIAN_POINT('Origin',(0.7,0.,15.3));
#14897=CARTESIAN_POINT('',(0.953939201416946,-0.3,15.3));
#14898=CARTESIAN_POINT('Ctrl Pts',(0.953939201416946,-0.3,15.3));
#14899=CARTESIAN_POINT('Ctrl Pts',(0.953939201416946,-0.3,15.3379277253989));
#14900=CARTESIAN_POINT('Ctrl Pts',(0.956437939057487,-0.292372091609923,
15.3782107485428));
#14901=CARTESIAN_POINT('Ctrl Pts',(0.965284956103207,-0.261686672615768,
15.4520475537716));
#14902=CARTESIAN_POINT('Ctrl Pts',(0.971486751729016,-0.238640531261463,
15.4856235374505));
#14903=CARTESIAN_POINT('Ctrl Pts',(0.982993562614982,-0.185631434471709,
15.5386326342402));
#14904=CARTESIAN_POINT('Ctrl Pts',(0.989071194990079,-0.152052241900624,
15.5616848907033));
#14905=CARTESIAN_POINT('Ctrl Pts',(0.997630133387832,-0.0782037717481885,
15.5923748246511));
#14906=CARTESIAN_POINT('Ctrl Pts',(1.,-0.0379164265292007,15.6));
#14907=CARTESIAN_POINT('Ctrl Pts',(1.,-2.70616862252382E-16,15.6));
#14908=CARTESIAN_POINT('',(0.7,-0.3,15.3));
#14909=CARTESIAN_POINT('',(0.7,-0.3,15.3));
#14910=CARTESIAN_POINT('Origin',(0.7,0.,15.3));
#14911=CARTESIAN_POINT('',(0.7,0.,15.6));
#14912=CARTESIAN_POINT('Origin',(0.7,0.3,13.7));
#14913=CARTESIAN_POINT('',(0.953939201416946,0.3,13.7));
#14914=CARTESIAN_POINT('',(0.953939201416946,0.3,-0.800000000000001));
#14915=CARTESIAN_POINT('',(0.7,0.3,13.7));
#14916=CARTESIAN_POINT('',(0.7,0.3,15.3));
#14917=CARTESIAN_POINT('',(0.7,0.3,13.7));
#14918=CARTESIAN_POINT('Origin',(0.7,0.,13.7));
#14919=CARTESIAN_POINT('',(0.953939201416946,-0.3,13.7));
#14920=CARTESIAN_POINT('Ctrl Pts',(0.953939201416946,0.3,13.7));
#14921=CARTESIAN_POINT('Ctrl Pts',(0.953939201416946,0.3,13.6620722746011));
#14922=CARTESIAN_POINT('Ctrl Pts',(0.956437939057488,0.292372091609922,
13.6217892514572));
#14923=CARTESIAN_POINT('Ctrl Pts',(0.965284956103208,0.261686672615766,
13.5479524462284));
#14924=CARTESIAN_POINT('Ctrl Pts',(0.971486751729016,0.238640531261462,
13.5143764625495));
#14925=CARTESIAN_POINT('Ctrl Pts',(0.982993562614982,0.185631434471708,
13.4613673657598));
#14926=CARTESIAN_POINT('Ctrl Pts',(0.98907119499008,0.152052241900622,13.4383151092967));
#14927=CARTESIAN_POINT('Ctrl Pts',(0.997630133387832,0.078203771748188,
13.4076251753489));
#14928=CARTESIAN_POINT('Ctrl Pts',(1.,0.0379164265292003,13.4));
#14929=CARTESIAN_POINT('Ctrl Pts',(1.,-0.0379164265292001,13.4));
#14930=CARTESIAN_POINT('Ctrl Pts',(0.997630133387832,-0.0782037717481879,
13.4076251753489));
#14931=CARTESIAN_POINT('Ctrl Pts',(0.98907119499008,-0.152052241900622,
13.4383151092967));
#14932=CARTESIAN_POINT('Ctrl Pts',(0.982993562614982,-0.185631434471708,
13.4613673657598));
#14933=CARTESIAN_POINT('Ctrl Pts',(0.971486751729016,-0.238640531261463,
13.5143764625495));
#14934=CARTESIAN_POINT('Ctrl Pts',(0.965284956103208,-0.261686672615766,
13.5479524462284));
#14935=CARTESIAN_POINT('Ctrl Pts',(0.956437939057488,-0.292372091609922,
13.6217892514572));
#14936=CARTESIAN_POINT('Ctrl Pts',(0.953939201416946,-0.3,13.6620722746011));
#14937=CARTESIAN_POINT('Ctrl Pts',(0.953939201416946,-0.3,13.7));
#14938=CARTESIAN_POINT('',(0.7,-0.3,13.7));
#14939=CARTESIAN_POINT('Origin',(0.7,0.,13.7));
#14940=CARTESIAN_POINT('',(0.7,-0.3,13.7));
#14941=CARTESIAN_POINT('Origin',(0.7,-0.3,15.3));
#14942=CARTESIAN_POINT('',(0.953939201416946,-0.3,-0.800000000000001));
#14943=CARTESIAN_POINT('',(0.7,-0.3,13.7));
#14944=CARTESIAN_POINT('Origin',(0.7,0.,14.5));
#14945=CARTESIAN_POINT('Origin',(0.,0.,-0.8));
#14946=CARTESIAN_POINT('',(-1.,-1.22464679914735E-16,15.6));
#14947=CARTESIAN_POINT('Origin',(0.,0.,15.6));
#14948=CARTESIAN_POINT('Origin',(0.,0.,15.6));
#14949=CARTESIAN_POINT('',(-1.,-1.22464679914735E-16,13.1));
#14950=CARTESIAN_POINT('',(-1.,-1.22464679914735E-16,-0.8));
#14951=CARTESIAN_POINT('Origin',(0.,0.,13.1));
#14952=CARTESIAN_POINT('Origin',(0.7,-0.3,6.9));
#14953=CARTESIAN_POINT('',(0.953939201416946,-0.3,6.3));
#14954=CARTESIAN_POINT('',(0.953939201416946,-0.3,6.9));
#14955=CARTESIAN_POINT('',(0.953939201416946,-0.3,-0.8));
#14956=CARTESIAN_POINT('',(0.7,-0.3,6.3));
#14957=CARTESIAN_POINT('',(0.7,-0.3,6.3));
#14958=CARTESIAN_POINT('',(0.7,-0.3,6.9));
#14959=CARTESIAN_POINT('',(0.7,-0.3,6.3));
#14960=CARTESIAN_POINT('',(0.7,-0.3,6.9));
#14961=CARTESIAN_POINT('Origin',(0.7,2.77555756156289E-17,6.9));
#14962=CARTESIAN_POINT('',(0.953939201416946,0.3,6.9));
#14963=CARTESIAN_POINT('Ctrl Pts',(0.953939201416946,-0.3,6.9));
#14964=CARTESIAN_POINT('Ctrl Pts',(0.953939201416946,-0.3,6.93792772539893));
#14965=CARTESIAN_POINT('Ctrl Pts',(0.956437939057488,-0.292372091609921,
6.97821074854282));
#14966=CARTESIAN_POINT('Ctrl Pts',(0.965284956103208,-0.261686672615765,
7.05204755377161));
#14967=CARTESIAN_POINT('Ctrl Pts',(0.971486751729016,-0.238640531261463,
7.08562353745047));
#14968=CARTESIAN_POINT('Ctrl Pts',(0.982993562614982,-0.185631434471708,
7.13863263424022));
#14969=CARTESIAN_POINT('Ctrl Pts',(0.98907119499008,-0.152052241900622,
7.1616848907033));
#14970=CARTESIAN_POINT('Ctrl Pts',(0.997630133387832,-0.078203771748188,
7.19237482465107));
#14971=CARTESIAN_POINT('Ctrl Pts',(1.,-0.0379164265292003,7.2));
#14972=CARTESIAN_POINT('Ctrl Pts',(1.,0.0379164265292002,7.2));
#14973=CARTESIAN_POINT('Ctrl Pts',(0.997630133387832,0.0782037717481879,
7.19237482465107));
#14974=CARTESIAN_POINT('Ctrl Pts',(0.98907119499008,0.152052241900622,7.1616848907033));
#14975=CARTESIAN_POINT('Ctrl Pts',(0.982993562614982,0.185631434471708,
7.13863263424022));
#14976=CARTESIAN_POINT('Ctrl Pts',(0.971486751729016,0.238640531261462,
7.08562353745047));
#14977=CARTESIAN_POINT('Ctrl Pts',(0.965284956103208,0.261686672615765,
7.05204755377162));
#14978=CARTESIAN_POINT('Ctrl Pts',(0.956437939057488,0.292372091609922,
6.97821074854282));
#14979=CARTESIAN_POINT('Ctrl Pts',(0.953939201416946,0.3,6.93792772539893));
#14980=CARTESIAN_POINT('Ctrl Pts',(0.953939201416946,0.3,6.9));
#14981=CARTESIAN_POINT('',(0.7,0.3,6.9));
#14982=CARTESIAN_POINT('Origin',(0.7,2.77555756156289E-17,6.9));
#14983=CARTESIAN_POINT('',(0.7,0.3,6.9));
#14984=CARTESIAN_POINT('Origin',(0.7,0.3,6.3));
#14985=CARTESIAN_POINT('',(0.953939201416946,0.3,6.3));
#14986=CARTESIAN_POINT('',(0.953939201416946,0.3,-0.8));
#14987=CARTESIAN_POINT('',(0.7,0.3,6.3));
#14988=CARTESIAN_POINT('',(0.7,0.3,6.9));
#14989=CARTESIAN_POINT('',(0.7,0.3,6.3));
#14990=CARTESIAN_POINT('Origin',(0.7,-2.77555756156289E-17,6.3));
#14991=CARTESIAN_POINT('Ctrl Pts',(0.953939201416946,0.3,6.3));
#14992=CARTESIAN_POINT('Ctrl Pts',(0.953939201416946,0.3,6.26207227460108));
#14993=CARTESIAN_POINT('Ctrl Pts',(0.956437939057488,0.292372091609921,
6.22178925145718));
#14994=CARTESIAN_POINT('Ctrl Pts',(0.965284956103208,0.261686672615765,
6.14795244622839));
#14995=CARTESIAN_POINT('Ctrl Pts',(0.971486751729016,0.238640531261462,
6.11437646254953));
#14996=CARTESIAN_POINT('Ctrl Pts',(0.982993562614982,0.185631434471708,
6.06136736575978));
#14997=CARTESIAN_POINT('Ctrl Pts',(0.98907119499008,0.152052241900622,6.0383151092967));
#14998=CARTESIAN_POINT('Ctrl Pts',(0.997630133387832,0.078203771748188,
6.00762517534893));
#14999=CARTESIAN_POINT('Ctrl Pts',(1.,0.0379164265292002,6.));
#15000=CARTESIAN_POINT('Ctrl Pts',(1.,-0.0379164265292002,6.));
#15001=CARTESIAN_POINT('Ctrl Pts',(0.997630133387832,-0.0782037717481879,
6.00762517534893));
#15002=CARTESIAN_POINT('Ctrl Pts',(0.98907119499008,-0.152052241900622,
6.0383151092967));
#15003=CARTESIAN_POINT('Ctrl Pts',(0.982993562614982,-0.185631434471708,
6.06136736575978));
#15004=CARTESIAN_POINT('Ctrl Pts',(0.971486751729016,-0.238640531261463,
6.11437646254953));
#15005=CARTESIAN_POINT('Ctrl Pts',(0.965284956103208,-0.261686672615765,
6.14795244622839));
#15006=CARTESIAN_POINT('Ctrl Pts',(0.956437939057488,-0.292372091609922,
6.22178925145718));
#15007=CARTESIAN_POINT('Ctrl Pts',(0.953939201416946,-0.3,6.26207227460108));
#15008=CARTESIAN_POINT('Ctrl Pts',(0.953939201416946,-0.3,6.3));
#15009=CARTESIAN_POINT('Origin',(0.7,-2.77555756156289E-17,6.3));
#15010=CARTESIAN_POINT('Origin',(0.7,0.,6.6));
#15011=CARTESIAN_POINT('Origin',(0.7,-0.3,2.7));
#15012=CARTESIAN_POINT('',(0.953939201416946,-0.3,2.1));
#15013=CARTESIAN_POINT('',(0.953939201416946,-0.3,2.7));
#15014=CARTESIAN_POINT('',(0.953939201416946,-0.3,-0.8));
#15015=CARTESIAN_POINT('',(0.7,-0.3,2.1));
#15016=CARTESIAN_POINT('',(0.7,-0.3,2.1));
#15017=CARTESIAN_POINT('',(0.7,-0.3,2.7));
#15018=CARTESIAN_POINT('',(0.7,-0.3,2.1));
#15019=CARTESIAN_POINT('',(0.7,-0.3,2.7));
#15020=CARTESIAN_POINT('Origin',(0.7,2.77555756156289E-17,2.7));
#15021=CARTESIAN_POINT('',(0.953939201416946,0.3,2.7));
#15022=CARTESIAN_POINT('Ctrl Pts',(0.953939201416946,-0.3,2.7));
#15023=CARTESIAN_POINT('Ctrl Pts',(0.953939201416946,-0.3,2.73792772539892));
#15024=CARTESIAN_POINT('Ctrl Pts',(0.956437939057488,-0.292372091609922,
2.77821074854282));
#15025=CARTESIAN_POINT('Ctrl Pts',(0.965284956103208,-0.261686672615765,
2.85204755377162));
#15026=CARTESIAN_POINT('Ctrl Pts',(0.971486751729016,-0.238640531261463,
2.88562353745047));
#15027=CARTESIAN_POINT('Ctrl Pts',(0.982993562614982,-0.185631434471708,
2.93863263424022));
#15028=CARTESIAN_POINT('Ctrl Pts',(0.98907119499008,-0.152052241900623,
2.9616848907033));
#15029=CARTESIAN_POINT('Ctrl Pts',(0.997630133387832,-0.078203771748188,
2.99237482465107));
#15030=CARTESIAN_POINT('Ctrl Pts',(1.,-0.0379164265292003,3.));
#15031=CARTESIAN_POINT('Ctrl Pts',(1.,0.0379164265292002,3.));
#15032=CARTESIAN_POINT('Ctrl Pts',(0.997630133387832,0.0782037717481883,
2.99237482465107));
#15033=CARTESIAN_POINT('Ctrl Pts',(0.98907119499008,0.152052241900623,2.9616848907033));
#15034=CARTESIAN_POINT('Ctrl Pts',(0.982993562614982,0.185631434471708,
2.93863263424022));
#15035=CARTESIAN_POINT('Ctrl Pts',(0.971486751729016,0.238640531261463,
2.88562353745047));
#15036=CARTESIAN_POINT('Ctrl Pts',(0.965284956103208,0.261686672615765,
2.85204755377162));
#15037=CARTESIAN_POINT('Ctrl Pts',(0.956437939057488,0.292372091609922,
2.77821074854282));
#15038=CARTESIAN_POINT('Ctrl Pts',(0.953939201416946,0.3,2.73792772539893));
#15039=CARTESIAN_POINT('Ctrl Pts',(0.953939201416946,0.3,2.7));
#15040=CARTESIAN_POINT('',(0.7,0.3,2.7));
#15041=CARTESIAN_POINT('Origin',(0.7,2.77555756156289E-17,2.7));
#15042=CARTESIAN_POINT('',(0.7,0.3,2.7));
#15043=CARTESIAN_POINT('Origin',(0.7,0.3,2.1));
#15044=CARTESIAN_POINT('',(0.953939201416946,0.3,2.1));
#15045=CARTESIAN_POINT('',(0.953939201416946,0.3,-0.8));
#15046=CARTESIAN_POINT('',(0.7,0.3,2.1));
#15047=CARTESIAN_POINT('',(0.7,0.3,2.7));
#15048=CARTESIAN_POINT('',(0.7,0.3,2.1));
#15049=CARTESIAN_POINT('Origin',(0.7,0.,2.1));
#15050=CARTESIAN_POINT('Ctrl Pts',(0.953939201416946,0.3,2.1));
#15051=CARTESIAN_POINT('Ctrl Pts',(0.953939201416946,0.3,2.06207227460107));
#15052=CARTESIAN_POINT('Ctrl Pts',(0.956437939057488,0.292372091609922,
2.02178925145718));
#15053=CARTESIAN_POINT('Ctrl Pts',(0.965284956103208,0.261686672615766,
1.94795244622839));
#15054=CARTESIAN_POINT('Ctrl Pts',(0.971486751729016,0.238640531261463,
1.91437646254953));
#15055=CARTESIAN_POINT('Ctrl Pts',(0.982993562614982,0.185631434471708,
1.86136736575978));
#15056=CARTESIAN_POINT('Ctrl Pts',(0.98907119499008,0.152052241900622,1.8383151092967));
#15057=CARTESIAN_POINT('Ctrl Pts',(0.997630133387832,0.0782037717481874,
1.80762517534893));
#15058=CARTESIAN_POINT('Ctrl Pts',(1.,0.0379164265292002,1.8));
#15059=CARTESIAN_POINT('Ctrl Pts',(1.,-0.0379164265292002,1.8));
#15060=CARTESIAN_POINT('Ctrl Pts',(0.997630133387832,-0.0782037717481877,
1.80762517534893));
#15061=CARTESIAN_POINT('Ctrl Pts',(0.98907119499008,-0.152052241900622,
1.8383151092967));
#15062=CARTESIAN_POINT('Ctrl Pts',(0.982993562614982,-0.185631434471708,
1.86136736575978));
#15063=CARTESIAN_POINT('Ctrl Pts',(0.971486751729016,-0.238640531261463,
1.91437646254953));
#15064=CARTESIAN_POINT('Ctrl Pts',(0.965284956103208,-0.261686672615765,
1.94795244622839));
#15065=CARTESIAN_POINT('Ctrl Pts',(0.956437939057488,-0.292372091609922,
2.02178925145718));
#15066=CARTESIAN_POINT('Ctrl Pts',(0.953939201416946,-0.3,2.06207227460107));
#15067=CARTESIAN_POINT('Ctrl Pts',(0.953939201416946,-0.3,2.1));
#15068=CARTESIAN_POINT('Origin',(0.7,0.,2.1));
#15069=CARTESIAN_POINT('Origin',(0.7,0.,2.4));
#15070=CARTESIAN_POINT('Origin',(0.,0.,13.05));
#15071=CARTESIAN_POINT('',(-0.9,-1.10218211923262E-16,13.));
#15072=CARTESIAN_POINT('Origin',(0.,0.,13.));
#15073=CARTESIAN_POINT('',(-0.9,-1.10218211923262E-16,13.1));
#15074=CARTESIAN_POINT('',(-0.9,-1.10218211923262E-16,13.05));
#15075=CARTESIAN_POINT('Origin',(0.,0.,13.1));
#15076=CARTESIAN_POINT('Origin',(1.3,0.,13.));
#15077=CARTESIAN_POINT('',(-1.,1.22464679914735E-16,13.));
#15078=CARTESIAN_POINT('Origin',(0.,0.,13.));
#15079=CARTESIAN_POINT('Origin',(0.9,0.,13.1));
#15080=CARTESIAN_POINT('Origin',(0.,0.,0.4));
#15081=CARTESIAN_POINT('',(-1.4,-1.71450551880629E-16,0.4));
#15082=CARTESIAN_POINT('Origin',(0.,0.,0.4));
#15083=CARTESIAN_POINT('',(-1.,-1.22464679914735E-16,0.4));
#15084=CARTESIAN_POINT('Origin',(0.,0.,0.4));
#15085=CARTESIAN_POINT('Origin',(0.,0.,0.));
#15086=CARTESIAN_POINT('',(-1.4,-1.71450551880629E-16,0.));
#15087=CARTESIAN_POINT('Origin',(0.,0.,0.));
#15088=CARTESIAN_POINT('',(-1.,1.22464679914735E-16,0.));
#15089=CARTESIAN_POINT('Origin',(0.,0.,0.));
#15090=CARTESIAN_POINT('Origin',(0.,0.,0.));
#15091=CARTESIAN_POINT('',(-1.4,-1.71450551880629E-16,0.));
#15092=CARTESIAN_POINT('Origin',(0.,0.,-0.8));
#15093=CARTESIAN_POINT('',(-1.,-1.22464679914735E-16,-0.8));
#15094=CARTESIAN_POINT('',(-1.,-1.22464679914735E-16,-0.8));
#15095=CARTESIAN_POINT('Origin',(0.,0.,-0.8));
#15096=CARTESIAN_POINT('Origin',(0.,0.,-0.8));
#15097=CARTESIAN_POINT('',(-1.,-1.22464679914735E-16,-0.8));
#15098=CARTESIAN_POINT('Origin',(0.,0.,15.6));
#15099=CARTESIAN_POINT('Origin',(0.,0.,-0.8));
#16654=UNCERTAINTY_MEASURE_WITH_UNIT(LENGTH_MEASURE(0.001),#16688,
'DISTANCE_ACCURACY_VALUE',
'Maximum model space distance between geometric entities at asserted c
onnectivities');
#16666=UNCERTAINTY_MEASURE_WITH_UNIT(LENGTH_MEASURE(0.001),#16688,
'DISTANCE_ACCURACY_VALUE',
'Maximum model space distance between geometric entities at asserted c
onnectivities');
#16675=(
GEOMETRIC_REPRESENTATION_CONTEXT(3)
GLOBAL_UNCERTAINTY_ASSIGNED_CONTEXT((#16654))
GLOBAL_UNIT_ASSIGNED_CONTEXT((#16688,#16690,#16691))
REPRESENTATION_CONTEXT('','3D')
);
#16687=(
GEOMETRIC_REPRESENTATION_CONTEXT(3)
GLOBAL_UNCERTAINTY_ASSIGNED_CONTEXT((#16666))
GLOBAL_UNIT_ASSIGNED_CONTEXT((#16688,#16690,#16691))
REPRESENTATION_CONTEXT('','3D')
);
#16688=(
LENGTH_UNIT()
NAMED_UNIT(*)
SI_UNIT(.CENTI.,.METRE.)
);
#16690=(
NAMED_UNIT(*)
PLANE_ANGLE_UNIT()
SI_UNIT($,.RADIAN.)
);
#16691=(
NAMED_UNIT(*)
SI_UNIT($,.STERADIAN.)
SOLID_ANGLE_UNIT()
);
#16700=SHAPE_DEFINITION_REPRESENTATION(#16720,#16771);
#16720=PRODUCT_DEFINITION_SHAPE('',$,#16792);
#16771=SHAPE_REPRESENTATION('',(#6778),#16675);
#16783=PRODUCT_DEFINITION_CONTEXT('part definition',#16845,'design');
#16792=PRODUCT_DEFINITION('Shaft','Shaft',#16812,#16783);
#16812=PRODUCT_DEFINITION_FORMATION('',$,#16855);
#16845=APPLICATION_CONTEXT(
'Core Data for Automotive Mechanical Design Process');
#16846=PRODUCT_CONTEXT('part definition',#16845,'mechanical');
#16855=PRODUCT('Shaft','Shaft','Shaft',(#16846));
#16873=PRESENTATION_STYLE_ASSIGNMENT((#16888));
#16888=SURFACE_STYLE_USAGE(.BOTH.,#16903);
#16903=SURFACE_SIDE_STYLE('',(#16918));
#16918=SURFACE_STYLE_FILL_AREA(#16933);
#16933=FILL_AREA_STYLE('Shaft gray',(#16948));
#16948=FILL_AREA_STYLE_COLOUR('Shaft gray',#16963);
#16963=COLOUR_RGB('Shaft gray',0.576470588235294,0.615686274509804,0.666666666666667);
ENDSEC;
END-ISO-10303-21;
